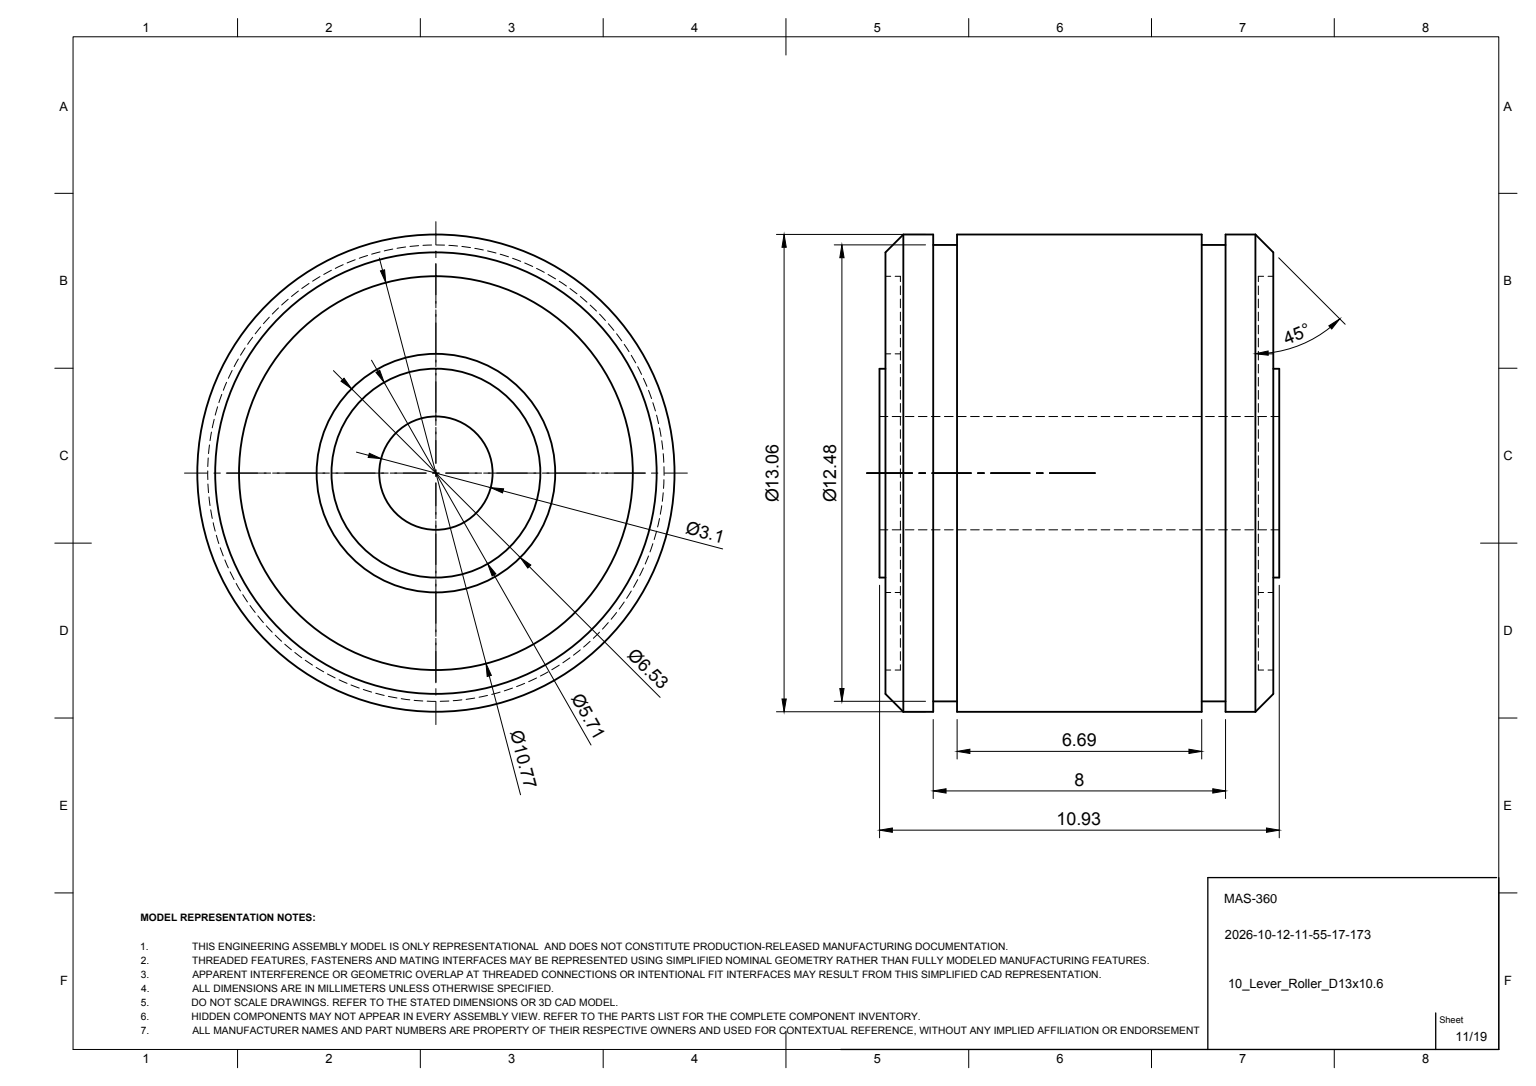
ISO-10303-21;
HEADER;
/* Generated by software containing ST-Developer
 * from STEP Tools, Inc. (www.steptools.com) 
 */

FILE_DESCRIPTION(
/* description */ (''),
/* implementation_level */ '2;1');

FILE_NAME(
/* name */ '10_Lever_Roller_D13x10.6.step',
/* time_stamp */ '2026-11-04T18:53:29-08:00',
/* author */ (''),
/* organization */ (''),
/* preprocessor_version */ 'ST-DEVELOPER v20.2',
/* originating_system */ 'Autodesk Translation Framework v15.17.0.0',
/* authorisation */ '');

FILE_SCHEMA (('AUTOMOTIVE_DESIGN { 1 0 10303 214 3 1 1 }'));
ENDSEC;

DATA;
#10=MECHANICAL_DESIGN_GEOMETRIC_PRESENTATION_REPRESENTATION('',(#1337),#100031);
#235=CONICAL_SURFACE('',#22396,6.2832,0.785398163397447);
#236=CONICAL_SURFACE('',#22400,6.2832,0.785398163397447);
#1116=CIRCLE('',#22353,2.8556);
#1117=CIRCLE('',#22354,1.55);
#1118=CIRCLE('',#22356,2.8556);
#1119=CIRCLE('',#22358,5.3856);
#1120=CIRCLE('',#22359,5.3856);
#1121=CIRCLE('',#22361,3.2636);
#1122=CIRCLE('',#22363,3.2636);
#1123=CIRCLE('',#22366,2.8556);
#1124=CIRCLE('',#22367,2.8556);
#1125=CIRCLE('',#22369,1.55);
#1126=CIRCLE('',#22371,3.2636);
#1127=CIRCLE('',#22372,3.2636);
#1128=CIRCLE('',#22374,5.3856);
#1129=CIRCLE('',#22376,5.3856);
#1130=CIRCLE('',#22378,6.0384);
#1131=CIRCLE('',#22380,6.528);
#1132=CIRCLE('',#22381,6.2424);
#1133=CIRCLE('',#22383,6.2424);
#1134=CIRCLE('',#22385,6.528);
#1135=CIRCLE('',#22387,6.528);
#1136=CIRCLE('',#22389,6.2424);
#1137=CIRCLE('',#22391,6.2424);
#1138=CIRCLE('',#22393,6.528);
#1139=CIRCLE('',#22395,6.528);
#1140=CIRCLE('',#22397,6.0384);
#1141=CIRCLE('',#22399,6.528);
#1301=SHAPE_REPRESENTATION_RELATIONSHIP('SRR','None',#100111,#1319);
#1319=ADVANCED_BREP_SHAPE_REPRESENTATION('',(#1355),#100023);
#1337=STYLED_ITEM('',(#100200),#1355);
#1355=MANIFOLD_SOLID_BREP('Body1',#20127);
#1663=PLANE('',#22352);
#1664=PLANE('',#22360);
#1665=PLANE('',#22364);
#1666=PLANE('',#22368);
#1667=PLANE('',#22373);
#1668=PLANE('',#22377);
#1669=PLANE('',#22379);
#1670=PLANE('',#22384);
#1671=PLANE('',#22388);
#1672=PLANE('',#22392);
#1673=PLANE('',#22401);
#1674=PLANE('',#22403);
#1790=FACE_BOUND('',#7364,.T.);
#1791=FACE_BOUND('',#7368,.T.);
#1792=FACE_BOUND('',#7371,.T.);
#1793=FACE_BOUND('',#7374,.T.);
#1794=FACE_BOUND('',#7377,.T.);
#1795=FACE_BOUND('',#7380,.T.);
#1796=FACE_BOUND('',#7382,.T.);
#1797=FACE_BOUND('',#7385,.T.);
#1798=FACE_BOUND('',#7388,.T.);
#1799=FACE_BOUND('',#7391,.T.);
#1800=FACE_BOUND('',#7397,.T.);
#1801=FACE_BOUND('',#7400,.T.);
#3227=LINE('',#99720,#4514);
#3228=LINE('',#99725,#4515);
#3229=LINE('',#99732,#4516);
#3230=LINE('',#99739,#4517);
#3231=LINE('',#99748,#4518);
#3232=LINE('',#99755,#4519);
#3233=LINE('',#99767,#4520);
#3234=LINE('',#99774,#4521);
#3235=LINE('',#99781,#4522);
#3236=LINE('',#99788,#4523);
#3237=LINE('',#99792,#4524);
#3238=LINE('',#99797,#4525);
#3239=LINE('',#99799,#4526);
#3240=LINE('',#99802,#4527);
#4514=VECTOR('',#27818,2.8556);
#4515=VECTOR('',#27823,5.3856);
#4516=VECTOR('',#27832,3.2636);
#4517=VECTOR('',#27841,2.8556);
#4518=VECTOR('',#27852,3.2636);
#4519=VECTOR('',#27861,5.3856);
#4520=VECTOR('',#27876,6.2424);
#4521=VECTOR('',#27885,6.528);
#4522=VECTOR('',#27894,6.2424);
#4523=VECTOR('',#27903,6.528);
#4524=VECTOR('',#27908,6.2832);
#4525=VECTOR('',#27915,6.528);
#4526=VECTOR('',#27918,6.2832);
#4527=VECTOR('',#27923,1.55);
#5001=CYLINDRICAL_SURFACE('',#22355,2.8556);
#5002=CYLINDRICAL_SURFACE('',#22357,5.3856);
#5003=CYLINDRICAL_SURFACE('',#22362,3.2636);
#5004=CYLINDRICAL_SURFACE('',#22365,2.8556);
#5005=CYLINDRICAL_SURFACE('',#22370,3.2636);
#5006=CYLINDRICAL_SURFACE('',#22375,5.3856);
#5007=CYLINDRICAL_SURFACE('',#22382,6.2424);
#5008=CYLINDRICAL_SURFACE('',#22386,6.528);
#5009=CYLINDRICAL_SURFACE('',#22390,6.2424);
#5010=CYLINDRICAL_SURFACE('',#22394,6.528);
#5011=CYLINDRICAL_SURFACE('',#22398,6.528);
#5012=CYLINDRICAL_SURFACE('',#22402,1.55);
#6110=FACE_OUTER_BOUND('',#7363,.T.);
#6111=FACE_OUTER_BOUND('',#7365,.T.);
#6112=FACE_OUTER_BOUND('',#7366,.T.);
#6113=FACE_OUTER_BOUND('',#7367,.T.);
#6114=FACE_OUTER_BOUND('',#7369,.T.);
#6115=FACE_OUTER_BOUND('',#7370,.T.);
#6116=FACE_OUTER_BOUND('',#7372,.T.);
#6117=FACE_OUTER_BOUND('',#7373,.T.);
#6118=FACE_OUTER_BOUND('',#7375,.T.);
#6119=FACE_OUTER_BOUND('',#7376,.T.);
#6120=FACE_OUTER_BOUND('',#7378,.T.);
#6121=FACE_OUTER_BOUND('',#7379,.T.);
#6122=FACE_OUTER_BOUND('',#7381,.T.);
#6123=FACE_OUTER_BOUND('',#7383,.T.);
#6124=FACE_OUTER_BOUND('',#7384,.T.);
#6125=FACE_OUTER_BOUND('',#7386,.T.);
#6126=FACE_OUTER_BOUND('',#7387,.T.);
#6127=FACE_OUTER_BOUND('',#7389,.T.);
#6128=FACE_OUTER_BOUND('',#7390,.T.);
#6129=FACE_OUTER_BOUND('',#7392,.T.);
#6130=FACE_OUTER_BOUND('',#7393,.T.);
#6131=FACE_OUTER_BOUND('',#7394,.T.);
#6132=FACE_OUTER_BOUND('',#7395,.T.);
#6133=FACE_OUTER_BOUND('',#7396,.T.);
#6134=FACE_OUTER_BOUND('',#7398,.T.);
#6135=FACE_OUTER_BOUND('',#7399,.T.);
#7363=EDGE_LOOP('',(#18635));
#7364=EDGE_LOOP('',(#18636));
#7365=EDGE_LOOP('',(#18637,#18638,#18639,#18640));
#7366=EDGE_LOOP('',(#18641,#18642,#18643,#18644));
#7367=EDGE_LOOP('',(#18645));
#7368=EDGE_LOOP('',(#18646));
#7369=EDGE_LOOP('',(#18647,#18648,#18649,#18650));
#7370=EDGE_LOOP('',(#18651));
#7371=EDGE_LOOP('',(#18652));
#7372=EDGE_LOOP('',(#18653,#18654,#18655,#18656));
#7373=EDGE_LOOP('',(#18657));
#7374=EDGE_LOOP('',(#18658));
#7375=EDGE_LOOP('',(#18659,#18660,#18661,#18662));
#7376=EDGE_LOOP('',(#18663));
#7377=EDGE_LOOP('',(#18664));
#7378=EDGE_LOOP('',(#18665,#18666,#18667,#18668));
#7379=EDGE_LOOP('',(#18669));
#7380=EDGE_LOOP('',(#18670));
#7381=EDGE_LOOP('',(#18671));
#7382=EDGE_LOOP('',(#18672));
#7383=EDGE_LOOP('',(#18673,#18674,#18675,#18676));
#7384=EDGE_LOOP('',(#18677));
#7385=EDGE_LOOP('',(#18678));
#7386=EDGE_LOOP('',(#18679,#18680,#18681,#18682));
#7387=EDGE_LOOP('',(#18683));
#7388=EDGE_LOOP('',(#18684));
#7389=EDGE_LOOP('',(#18685,#18686,#18687,#18688));
#7390=EDGE_LOOP('',(#18689));
#7391=EDGE_LOOP('',(#18690));
#7392=EDGE_LOOP('',(#18691,#18692,#18693,#18694));
#7393=EDGE_LOOP('',(#18695,#18696,#18697,#18698));
#7394=EDGE_LOOP('',(#18699,#18700,#18701,#18702));
#7395=EDGE_LOOP('',(#18703,#18704,#18705,#18706));
#7396=EDGE_LOOP('',(#18707));
#7397=EDGE_LOOP('',(#18708));
#7398=EDGE_LOOP('',(#18709,#18710,#18711,#18712));
#7399=EDGE_LOOP('',(#18713));
#7400=EDGE_LOOP('',(#18714));
#9857=VERTEX_POINT('',#99713);
#9858=VERTEX_POINT('',#99715);
#9859=VERTEX_POINT('',#99718);
#9860=VERTEX_POINT('',#99722);
#9861=VERTEX_POINT('',#99724);
#9862=VERTEX_POINT('',#99728);
#9863=VERTEX_POINT('',#99731);
#9864=VERTEX_POINT('',#99736);
#9865=VERTEX_POINT('',#99738);
#9866=VERTEX_POINT('',#99742);
#9867=VERTEX_POINT('',#99745);
#9868=VERTEX_POINT('',#99747);
#9869=VERTEX_POINT('',#99751);
#9870=VERTEX_POINT('',#99754);
#9871=VERTEX_POINT('',#99758);
#9872=VERTEX_POINT('',#99761);
#9873=VERTEX_POINT('',#99763);
#9874=VERTEX_POINT('',#99766);
#9875=VERTEX_POINT('',#99770);
#9876=VERTEX_POINT('',#99773);
#9877=VERTEX_POINT('',#99777);
#9878=VERTEX_POINT('',#99780);
#9879=VERTEX_POINT('',#99784);
#9880=VERTEX_POINT('',#99787);
#9881=VERTEX_POINT('',#99791);
#9882=VERTEX_POINT('',#99795);
#12792=EDGE_CURVE('',#9857,#9857,#1116,.T.);
#12793=EDGE_CURVE('',#9858,#9858,#1117,.T.);
#12794=EDGE_CURVE('',#9859,#9859,#1118,.T.);
#12795=EDGE_CURVE('',#9859,#9857,#3227,.T.);
#12796=EDGE_CURVE('',#9860,#9860,#1119,.T.);
#12797=EDGE_CURVE('',#9860,#9861,#3228,.T.);
#12798=EDGE_CURVE('',#9861,#9861,#1120,.T.);
#12799=EDGE_CURVE('',#9862,#9862,#1121,.T.);
#12800=EDGE_CURVE('',#9862,#9863,#3229,.T.);
#12801=EDGE_CURVE('',#9863,#9863,#1122,.T.);
#12802=EDGE_CURVE('',#9864,#9864,#1123,.T.);
#12803=EDGE_CURVE('',#9864,#9865,#3230,.T.);
#12804=EDGE_CURVE('',#9865,#9865,#1124,.T.);
#12805=EDGE_CURVE('',#9866,#9866,#1125,.T.);
#12806=EDGE_CURVE('',#9867,#9867,#1126,.T.);
#12807=EDGE_CURVE('',#9867,#9868,#3231,.T.);
#12808=EDGE_CURVE('',#9868,#9868,#1127,.T.);
#12809=EDGE_CURVE('',#9869,#9869,#1128,.T.);
#12810=EDGE_CURVE('',#9869,#9870,#3232,.T.);
#12811=EDGE_CURVE('',#9870,#9870,#1129,.T.);
#12812=EDGE_CURVE('',#9871,#9871,#1130,.T.);
#12813=EDGE_CURVE('',#9872,#9872,#1131,.T.);
#12814=EDGE_CURVE('',#9873,#9873,#1132,.T.);
#12815=EDGE_CURVE('',#9873,#9874,#3233,.T.);
#12816=EDGE_CURVE('',#9874,#9874,#1133,.T.);
#12817=EDGE_CURVE('',#9875,#9875,#1134,.T.);
#12818=EDGE_CURVE('',#9875,#9876,#3234,.T.);
#12819=EDGE_CURVE('',#9876,#9876,#1135,.T.);
#12820=EDGE_CURVE('',#9877,#9877,#1136,.T.);
#12821=EDGE_CURVE('',#9877,#9878,#3235,.T.);
#12822=EDGE_CURVE('',#9878,#9878,#1137,.T.);
#12823=EDGE_CURVE('',#9879,#9879,#1138,.T.);
#12824=EDGE_CURVE('',#9879,#9880,#3236,.T.);
#12825=EDGE_CURVE('',#9880,#9880,#1139,.T.);
#12826=EDGE_CURVE('',#9880,#9881,#3237,.T.);
#12827=EDGE_CURVE('',#9881,#9881,#1140,.T.);
#12828=EDGE_CURVE('',#9882,#9882,#1141,.T.);
#12829=EDGE_CURVE('',#9882,#9872,#3238,.T.);
#12830=EDGE_CURVE('',#9882,#9871,#3239,.T.);
#12831=EDGE_CURVE('',#9858,#9866,#3240,.T.);
#18635=ORIENTED_EDGE('',*,*,#12792,.F.);
#18636=ORIENTED_EDGE('',*,*,#12793,.T.);
#18637=ORIENTED_EDGE('',*,*,#12794,.F.);
#18638=ORIENTED_EDGE('',*,*,#12795,.T.);
#18639=ORIENTED_EDGE('',*,*,#12792,.T.);
#18640=ORIENTED_EDGE('',*,*,#12795,.F.);
#18641=ORIENTED_EDGE('',*,*,#12796,.F.);
#18642=ORIENTED_EDGE('',*,*,#12797,.T.);
#18643=ORIENTED_EDGE('',*,*,#12798,.T.);
#18644=ORIENTED_EDGE('',*,*,#12797,.F.);
#18645=ORIENTED_EDGE('',*,*,#12798,.F.);
#18646=ORIENTED_EDGE('',*,*,#12799,.T.);
#18647=ORIENTED_EDGE('',*,*,#12799,.F.);
#18648=ORIENTED_EDGE('',*,*,#12800,.T.);
#18649=ORIENTED_EDGE('',*,*,#12801,.F.);
#18650=ORIENTED_EDGE('',*,*,#12800,.F.);
#18651=ORIENTED_EDGE('',*,*,#12801,.T.);
#18652=ORIENTED_EDGE('',*,*,#12794,.T.);
#18653=ORIENTED_EDGE('',*,*,#12802,.F.);
#18654=ORIENTED_EDGE('',*,*,#12803,.T.);
#18655=ORIENTED_EDGE('',*,*,#12804,.F.);
#18656=ORIENTED_EDGE('',*,*,#12803,.F.);
#18657=ORIENTED_EDGE('',*,*,#12802,.T.);
#18658=ORIENTED_EDGE('',*,*,#12805,.F.);
#18659=ORIENTED_EDGE('',*,*,#12806,.F.);
#18660=ORIENTED_EDGE('',*,*,#12807,.T.);
#18661=ORIENTED_EDGE('',*,*,#12808,.T.);
#18662=ORIENTED_EDGE('',*,*,#12807,.F.);
#18663=ORIENTED_EDGE('',*,*,#12809,.T.);
#18664=ORIENTED_EDGE('',*,*,#12808,.F.);
#18665=ORIENTED_EDGE('',*,*,#12809,.F.);
#18666=ORIENTED_EDGE('',*,*,#12810,.T.);
#18667=ORIENTED_EDGE('',*,*,#12811,.F.);
#18668=ORIENTED_EDGE('',*,*,#12810,.F.);
#18669=ORIENTED_EDGE('',*,*,#12812,.T.);
#18670=ORIENTED_EDGE('',*,*,#12811,.T.);
#18671=ORIENTED_EDGE('',*,*,#12813,.F.);
#18672=ORIENTED_EDGE('',*,*,#12814,.T.);
#18673=ORIENTED_EDGE('',*,*,#12814,.F.);
#18674=ORIENTED_EDGE('',*,*,#12815,.T.);
#18675=ORIENTED_EDGE('',*,*,#12816,.T.);
#18676=ORIENTED_EDGE('',*,*,#12815,.F.);
#18677=ORIENTED_EDGE('',*,*,#12817,.F.);
#18678=ORIENTED_EDGE('',*,*,#12816,.F.);
#18679=ORIENTED_EDGE('',*,*,#12817,.T.);
#18680=ORIENTED_EDGE('',*,*,#12818,.T.);
#18681=ORIENTED_EDGE('',*,*,#12819,.T.);
#18682=ORIENTED_EDGE('',*,*,#12818,.F.);
#18683=ORIENTED_EDGE('',*,*,#12819,.F.);
#18684=ORIENTED_EDGE('',*,*,#12820,.T.);
#18685=ORIENTED_EDGE('',*,*,#12820,.F.);
#18686=ORIENTED_EDGE('',*,*,#12821,.T.);
#18687=ORIENTED_EDGE('',*,*,#12822,.T.);
#18688=ORIENTED_EDGE('',*,*,#12821,.F.);
#18689=ORIENTED_EDGE('',*,*,#12823,.F.);
#18690=ORIENTED_EDGE('',*,*,#12822,.F.);
#18691=ORIENTED_EDGE('',*,*,#12823,.T.);
#18692=ORIENTED_EDGE('',*,*,#12824,.T.);
#18693=ORIENTED_EDGE('',*,*,#12825,.T.);
#18694=ORIENTED_EDGE('',*,*,#12824,.F.);
#18695=ORIENTED_EDGE('',*,*,#12825,.F.);
#18696=ORIENTED_EDGE('',*,*,#12826,.T.);
#18697=ORIENTED_EDGE('',*,*,#12827,.T.);
#18698=ORIENTED_EDGE('',*,*,#12826,.F.);
#18699=ORIENTED_EDGE('',*,*,#12828,.F.);
#18700=ORIENTED_EDGE('',*,*,#12829,.T.);
#18701=ORIENTED_EDGE('',*,*,#12813,.T.);
#18702=ORIENTED_EDGE('',*,*,#12829,.F.);
#18703=ORIENTED_EDGE('',*,*,#12828,.T.);
#18704=ORIENTED_EDGE('',*,*,#12830,.T.);
#18705=ORIENTED_EDGE('',*,*,#12812,.F.);
#18706=ORIENTED_EDGE('',*,*,#12830,.F.);
#18707=ORIENTED_EDGE('',*,*,#12806,.T.);
#18708=ORIENTED_EDGE('',*,*,#12804,.T.);
#18709=ORIENTED_EDGE('',*,*,#12793,.F.);
#18710=ORIENTED_EDGE('',*,*,#12831,.T.);
#18711=ORIENTED_EDGE('',*,*,#12805,.T.);
#18712=ORIENTED_EDGE('',*,*,#12831,.F.);
#18713=ORIENTED_EDGE('',*,*,#12827,.F.);
#18714=ORIENTED_EDGE('',*,*,#12796,.T.);
#20044=ADVANCED_FACE('',(#6110,#1790),#1663,.T.);
#20045=ADVANCED_FACE('',(#6111),#5001,.T.);
#20046=ADVANCED_FACE('',(#6112),#5002,.F.);
#20047=ADVANCED_FACE('',(#6113,#1791),#1664,.F.);
#20048=ADVANCED_FACE('',(#6114),#5003,.T.);
#20049=ADVANCED_FACE('',(#6115,#1792),#1665,.T.);
#20050=ADVANCED_FACE('',(#6116),#5004,.T.);
#20051=ADVANCED_FACE('',(#6117,#1793),#1666,.T.);
#20052=ADVANCED_FACE('',(#6118),#5005,.T.);
#20053=ADVANCED_FACE('',(#6119,#1794),#1667,.F.);
#20054=ADVANCED_FACE('',(#6120),#5006,.F.);
#20055=ADVANCED_FACE('',(#6121,#1795),#1668,.T.);
#20056=ADVANCED_FACE('',(#6122,#1796),#1669,.F.);
#20057=ADVANCED_FACE('',(#6123),#5007,.T.);
#20058=ADVANCED_FACE('',(#6124,#1797),#1670,.F.);
#20059=ADVANCED_FACE('',(#6125),#5008,.T.);
#20060=ADVANCED_FACE('',(#6126,#1798),#1671,.F.);
#20061=ADVANCED_FACE('',(#6127),#5009,.T.);
#20062=ADVANCED_FACE('',(#6128,#1799),#1672,.F.);
#20063=ADVANCED_FACE('',(#6129),#5010,.T.);
#20064=ADVANCED_FACE('',(#6130),#235,.T.);
#20065=ADVANCED_FACE('',(#6131),#5011,.T.);
#20066=ADVANCED_FACE('',(#6132),#236,.T.);
#20067=ADVANCED_FACE('',(#6133,#1800),#1673,.T.);
#20068=ADVANCED_FACE('',(#6134),#5012,.F.);
#20069=ADVANCED_FACE('',(#6135,#1801),#1674,.T.);
#20127=CLOSED_SHELL('',(#20044,#20045,#20046,#20047,#20048,#20049,#20050,
#20051,#20052,#20053,#20054,#20055,#20056,#20057,#20058,#20059,#20060,#20061,
#20062,#20063,#20064,#20065,#20066,#20067,#20068,#20069));
#22351=AXIS2_PLACEMENT_3D('',#99711,#27806,#27807);
#22352=AXIS2_PLACEMENT_3D('',#99712,#27808,#27809);
#22353=AXIS2_PLACEMENT_3D('',#99714,#27810,#27811);
#22354=AXIS2_PLACEMENT_3D('',#99716,#27812,#27813);
#22355=AXIS2_PLACEMENT_3D('',#99717,#27814,#27815);
#22356=AXIS2_PLACEMENT_3D('',#99719,#27816,#27817);
#22357=AXIS2_PLACEMENT_3D('',#99721,#27819,#27820);
#22358=AXIS2_PLACEMENT_3D('',#99723,#27821,#27822);
#22359=AXIS2_PLACEMENT_3D('',#99726,#27824,#27825);
#22360=AXIS2_PLACEMENT_3D('',#99727,#27826,#27827);
#22361=AXIS2_PLACEMENT_3D('',#99729,#27828,#27829);
#22362=AXIS2_PLACEMENT_3D('',#99730,#27830,#27831);
#22363=AXIS2_PLACEMENT_3D('',#99733,#27833,#27834);
#22364=AXIS2_PLACEMENT_3D('',#99734,#27835,#27836);
#22365=AXIS2_PLACEMENT_3D('',#99735,#27837,#27838);
#22366=AXIS2_PLACEMENT_3D('',#99737,#27839,#27840);
#22367=AXIS2_PLACEMENT_3D('',#99740,#27842,#27843);
#22368=AXIS2_PLACEMENT_3D('',#99741,#27844,#27845);
#22369=AXIS2_PLACEMENT_3D('',#99743,#27846,#27847);
#22370=AXIS2_PLACEMENT_3D('',#99744,#27848,#27849);
#22371=AXIS2_PLACEMENT_3D('',#99746,#27850,#27851);
#22372=AXIS2_PLACEMENT_3D('',#99749,#27853,#27854);
#22373=AXIS2_PLACEMENT_3D('',#99750,#27855,#27856);
#22374=AXIS2_PLACEMENT_3D('',#99752,#27857,#27858);
#22375=AXIS2_PLACEMENT_3D('',#99753,#27859,#27860);
#22376=AXIS2_PLACEMENT_3D('',#99756,#27862,#27863);
#22377=AXIS2_PLACEMENT_3D('',#99757,#27864,#27865);
#22378=AXIS2_PLACEMENT_3D('',#99759,#27866,#27867);
#22379=AXIS2_PLACEMENT_3D('',#99760,#27868,#27869);
#22380=AXIS2_PLACEMENT_3D('',#99762,#27870,#27871);
#22381=AXIS2_PLACEMENT_3D('',#99764,#27872,#27873);
#22382=AXIS2_PLACEMENT_3D('',#99765,#27874,#27875);
#22383=AXIS2_PLACEMENT_3D('',#99768,#27877,#27878);
#22384=AXIS2_PLACEMENT_3D('',#99769,#27879,#27880);
#22385=AXIS2_PLACEMENT_3D('',#99771,#27881,#27882);
#22386=AXIS2_PLACEMENT_3D('',#99772,#27883,#27884);
#22387=AXIS2_PLACEMENT_3D('',#99775,#27886,#27887);
#22388=AXIS2_PLACEMENT_3D('',#99776,#27888,#27889);
#22389=AXIS2_PLACEMENT_3D('',#99778,#27890,#27891);
#22390=AXIS2_PLACEMENT_3D('',#99779,#27892,#27893);
#22391=AXIS2_PLACEMENT_3D('',#99782,#27895,#27896);
#22392=AXIS2_PLACEMENT_3D('',#99783,#27897,#27898);
#22393=AXIS2_PLACEMENT_3D('',#99785,#27899,#27900);
#22394=AXIS2_PLACEMENT_3D('',#99786,#27901,#27902);
#22395=AXIS2_PLACEMENT_3D('',#99789,#27904,#27905);
#22396=AXIS2_PLACEMENT_3D('',#99790,#27906,#27907);
#22397=AXIS2_PLACEMENT_3D('',#99793,#27909,#27910);
#22398=AXIS2_PLACEMENT_3D('',#99794,#27911,#27912);
#22399=AXIS2_PLACEMENT_3D('',#99796,#27913,#27914);
#22400=AXIS2_PLACEMENT_3D('',#99798,#27916,#27917);
#22401=AXIS2_PLACEMENT_3D('',#99800,#27919,#27920);
#22402=AXIS2_PLACEMENT_3D('',#99801,#27921,#27922);
#22403=AXIS2_PLACEMENT_3D('',#99803,#27924,#27925);
#27806=DIRECTION('axis',(0.,0.,1.));
#27807=DIRECTION('refdir',(1.,0.,0.));
#27808=DIRECTION('center_axis',(-1.,0.,0.));
#27809=DIRECTION('ref_axis',(0.,0.,1.));
#27810=DIRECTION('center_axis',(1.,0.,0.));
#27811=DIRECTION('ref_axis',(0.,0.,-1.));
#27812=DIRECTION('center_axis',(1.,0.,0.));
#27813=DIRECTION('ref_axis',(0.,0.,-1.));
#27814=DIRECTION('center_axis',(1.,0.,0.));
#27815=DIRECTION('ref_axis',(0.,1.,0.));
#27816=DIRECTION('center_axis',(1.,0.,0.));
#27817=DIRECTION('ref_axis',(0.,1.,0.));
#27818=DIRECTION('',(-1.,0.,0.));
#27819=DIRECTION('center_axis',(1.,0.,0.));
#27820=DIRECTION('ref_axis',(0.,1.,0.));
#27821=DIRECTION('center_axis',(1.,0.,0.));
#27822=DIRECTION('ref_axis',(0.,1.,0.));
#27823=DIRECTION('',(1.,0.,0.));
#27824=DIRECTION('center_axis',(1.,0.,0.));
#27825=DIRECTION('ref_axis',(0.,0.,-1.));
#27826=DIRECTION('center_axis',(1.,0.,0.));
#27827=DIRECTION('ref_axis',(0.,0.,-1.));
#27828=DIRECTION('center_axis',(1.,0.,0.));
#27829=DIRECTION('ref_axis',(0.,0.,-1.));
#27830=DIRECTION('center_axis',(1.,0.,0.));
#27831=DIRECTION('ref_axis',(0.,1.,0.));
#27832=DIRECTION('',(-1.,0.,0.));
#27833=DIRECTION('center_axis',(-1.,0.,0.));
#27834=DIRECTION('ref_axis',(0.,1.,0.));
#27835=DIRECTION('center_axis',(-1.,0.,0.));
#27836=DIRECTION('ref_axis',(0.,0.,1.));
#27837=DIRECTION('center_axis',(1.,0.,0.));
#27838=DIRECTION('ref_axis',(0.,1.,0.));
#27839=DIRECTION('center_axis',(1.,0.,0.));
#27840=DIRECTION('ref_axis',(0.,0.,-1.));
#27841=DIRECTION('',(-1.,0.,0.));
#27842=DIRECTION('center_axis',(-1.,0.,0.));
#27843=DIRECTION('ref_axis',(0.,1.,0.));
#27844=DIRECTION('center_axis',(1.,0.,0.));
#27845=DIRECTION('ref_axis',(0.,0.,-1.));
#27846=DIRECTION('center_axis',(1.,0.,0.));
#27847=DIRECTION('ref_axis',(0.,0.,-1.));
#27848=DIRECTION('center_axis',(1.,0.,0.));
#27849=DIRECTION('ref_axis',(0.,1.,0.));
#27850=DIRECTION('center_axis',(1.,0.,0.));
#27851=DIRECTION('ref_axis',(0.,1.,0.));
#27852=DIRECTION('',(-1.,0.,0.));
#27853=DIRECTION('center_axis',(1.,0.,0.));
#27854=DIRECTION('ref_axis',(0.,0.,-1.));
#27855=DIRECTION('center_axis',(-1.,0.,0.));
#27856=DIRECTION('ref_axis',(0.,0.,1.));
#27857=DIRECTION('center_axis',(1.,0.,0.));
#27858=DIRECTION('ref_axis',(0.,0.,-1.));
#27859=DIRECTION('center_axis',(1.,0.,0.));
#27860=DIRECTION('ref_axis',(0.,1.,0.));
#27861=DIRECTION('',(1.,0.,0.));
#27862=DIRECTION('center_axis',(-1.,0.,0.));
#27863=DIRECTION('ref_axis',(0.,1.,0.));
#27864=DIRECTION('center_axis',(1.,0.,0.));
#27865=DIRECTION('ref_axis',(0.,0.,-1.));
#27866=DIRECTION('center_axis',(1.,0.,0.));
#27867=DIRECTION('ref_axis',(0.,0.,-1.));
#27868=DIRECTION('center_axis',(1.,0.,0.));
#27869=DIRECTION('ref_axis',(0.,0.,-1.));
#27870=DIRECTION('center_axis',(1.,0.,0.));
#27871=DIRECTION('ref_axis',(0.,1.,0.));
#27872=DIRECTION('center_axis',(1.,0.,0.));
#27873=DIRECTION('ref_axis',(0.,0.,-1.));
#27874=DIRECTION('center_axis',(1.,0.,0.));
#27875=DIRECTION('ref_axis',(0.,1.,0.));
#27876=DIRECTION('',(-1.,0.,0.));
#27877=DIRECTION('center_axis',(1.,0.,0.));
#27878=DIRECTION('ref_axis',(0.,0.,-1.));
#27879=DIRECTION('center_axis',(-1.,0.,0.));
#27880=DIRECTION('ref_axis',(0.,0.,1.));
#27881=DIRECTION('center_axis',(-1.,0.,0.));
#27882=DIRECTION('ref_axis',(0.,1.,0.));
#27883=DIRECTION('center_axis',(1.,0.,0.));
#27884=DIRECTION('ref_axis',(0.,1.,0.));
#27885=DIRECTION('',(-1.,0.,0.));
#27886=DIRECTION('center_axis',(1.,0.,0.));
#27887=DIRECTION('ref_axis',(0.,1.,0.));
#27888=DIRECTION('center_axis',(1.,0.,0.));
#27889=DIRECTION('ref_axis',(0.,0.,-1.));
#27890=DIRECTION('center_axis',(1.,0.,0.));
#27891=DIRECTION('ref_axis',(0.,0.,-1.));
#27892=DIRECTION('center_axis',(1.,0.,0.));
#27893=DIRECTION('ref_axis',(0.,1.,0.));
#27894=DIRECTION('',(-1.,0.,0.));
#27895=DIRECTION('center_axis',(1.,0.,0.));
#27896=DIRECTION('ref_axis',(0.,0.,-1.));
#27897=DIRECTION('center_axis',(-1.,0.,0.));
#27898=DIRECTION('ref_axis',(0.,0.,1.));
#27899=DIRECTION('center_axis',(-1.,0.,0.));
#27900=DIRECTION('ref_axis',(0.,1.,0.));
#27901=DIRECTION('center_axis',(1.,0.,0.));
#27902=DIRECTION('ref_axis',(0.,1.,0.));
#27903=DIRECTION('',(-1.,0.,0.));
#27904=DIRECTION('center_axis',(1.,0.,0.));
#27905=DIRECTION('ref_axis',(0.,0.,-1.));
#27906=DIRECTION('center_axis',(1.,0.,0.));
#27907=DIRECTION('ref_axis',(0.,1.,0.));
#27908=DIRECTION('',(-0.707106781186548,0.707106781186547,8.65956056235492E-17));
#27909=DIRECTION('center_axis',(1.,0.,0.));
#27910=DIRECTION('ref_axis',(0.,0.,-1.));
#27911=DIRECTION('center_axis',(1.,0.,0.));
#27912=DIRECTION('ref_axis',(0.,1.,0.));
#27913=DIRECTION('center_axis',(1.,0.,0.));
#27914=DIRECTION('ref_axis',(0.,0.,-1.));
#27915=DIRECTION('',(-1.,0.,0.));
#27916=DIRECTION('center_axis',(-1.,0.,0.));
#27917=DIRECTION('ref_axis',(0.,1.,0.));
#27918=DIRECTION('',(0.707106781186548,0.707106781186547,-8.65956056235492E-17));
#27919=DIRECTION('center_axis',(1.,0.,0.));
#27920=DIRECTION('ref_axis',(0.,0.,-1.));
#27921=DIRECTION('center_axis',(1.,0.,0.));
#27922=DIRECTION('ref_axis',(0.,1.,0.));
#27923=DIRECTION('',(1.,0.,0.));
#27924=DIRECTION('center_axis',(-1.,0.,0.));
#27925=DIRECTION('ref_axis',(0.,0.,1.));
#99711=CARTESIAN_POINT('',(0.,0.,0.));
#99712=CARTESIAN_POINT('Origin',(-5.4672,2.8556,0.));
#99713=CARTESIAN_POINT('',(-5.4672,-2.8556,-3.49710139964518E-16));
#99714=CARTESIAN_POINT('Origin',(-5.4672,0.,0.));
#99715=CARTESIAN_POINT('',(-5.4672,-1.55,-1.8982025386784E-16));
#99716=CARTESIAN_POINT('Origin',(-5.4672,0.,0.));
#99717=CARTESIAN_POINT('Origin',(-5.3856,0.,0.));
#99718=CARTESIAN_POINT('',(-5.304,-2.8556,-3.49710139964518E-16));
#99719=CARTESIAN_POINT('Origin',(-5.304,0.,0.));
#99720=CARTESIAN_POINT('',(-5.3856,-2.8556,-3.49710139964518E-16));
#99721=CARTESIAN_POINT('Origin',(-5.1,0.,0.));
#99722=CARTESIAN_POINT('',(-5.304,-5.3856,-6.59545780148798E-16));
#99723=CARTESIAN_POINT('Origin',(-5.304,0.,0.));
#99724=CARTESIAN_POINT('',(-4.896,-5.3856,-6.59545780148798E-16));
#99725=CARTESIAN_POINT('',(-5.1,-5.3856,-6.59545780148799E-16));
#99726=CARTESIAN_POINT('Origin',(-4.896,0.,0.));
#99727=CARTESIAN_POINT('Origin',(-4.896,3.2636,0.));
#99728=CARTESIAN_POINT('',(-4.896,-3.2636,-3.9967572936973E-16));
#99729=CARTESIAN_POINT('Origin',(-4.896,0.,0.));
#99730=CARTESIAN_POINT('Origin',(-5.1,0.,0.));
#99731=CARTESIAN_POINT('',(-5.304,-3.2636,-3.9967572936973E-16));
#99732=CARTESIAN_POINT('',(-5.1,-3.2636,-3.9967572936973E-16));
#99733=CARTESIAN_POINT('Origin',(-5.304,0.,0.));
#99734=CARTESIAN_POINT('Origin',(-5.304,6.0384,0.));
#99735=CARTESIAN_POINT('Origin',(5.3856,0.,0.));
#99736=CARTESIAN_POINT('',(5.4672,-2.8556,-3.49710139964518E-16));
#99737=CARTESIAN_POINT('Origin',(5.4672,0.,0.));
#99738=CARTESIAN_POINT('',(5.304,-2.8556,-3.49710139964518E-16));
#99739=CARTESIAN_POINT('',(5.3856,-2.8556,-3.49710139964518E-16));
#99740=CARTESIAN_POINT('Origin',(5.304,0.,0.));
#99741=CARTESIAN_POINT('Origin',(5.4672,1.55,0.));
#99742=CARTESIAN_POINT('',(5.4672,-1.55,-1.8982025386784E-16));
#99743=CARTESIAN_POINT('Origin',(5.4672,0.,0.));
#99744=CARTESIAN_POINT('Origin',(5.1,0.,0.));
#99745=CARTESIAN_POINT('',(5.304,-3.2636,-3.9967572936973E-16));
#99746=CARTESIAN_POINT('Origin',(5.304,0.,0.));
#99747=CARTESIAN_POINT('',(4.896,-3.2636,-3.9967572936973E-16));
#99748=CARTESIAN_POINT('',(5.1,-3.2636,-3.9967572936973E-16));
#99749=CARTESIAN_POINT('Origin',(4.896,0.,0.));
#99750=CARTESIAN_POINT('Origin',(4.896,5.3856,0.));
#99751=CARTESIAN_POINT('',(4.896,-5.3856,-6.59545780148798E-16));
#99752=CARTESIAN_POINT('Origin',(4.896,0.,0.));
#99753=CARTESIAN_POINT('Origin',(5.1,0.,0.));
#99754=CARTESIAN_POINT('',(5.304,-5.3856,-6.59545780148798E-16));
#99755=CARTESIAN_POINT('',(5.1,-5.3856,-6.59545780148799E-16));
#99756=CARTESIAN_POINT('Origin',(5.304,0.,0.));
#99757=CARTESIAN_POINT('Origin',(5.304,1.55,0.));
#99758=CARTESIAN_POINT('',(5.304,-6.0384,-7.39490723197138E-16));
#99759=CARTESIAN_POINT('Origin',(5.304,0.,0.));
#99760=CARTESIAN_POINT('Origin',(3.9984,6.2424,0.));
#99761=CARTESIAN_POINT('',(3.9984,-6.528,-7.99449430483392E-16));
#99762=CARTESIAN_POINT('Origin',(3.9984,0.,0.));
#99763=CARTESIAN_POINT('',(3.9984,-6.2424,-7.64473517899744E-16));
#99764=CARTESIAN_POINT('Origin',(3.9984,0.,0.));
#99765=CARTESIAN_POINT('Origin',(3.672,0.,0.));
#99766=CARTESIAN_POINT('',(3.3456,-6.2424,-7.64473517899744E-16));
#99767=CARTESIAN_POINT('',(3.672,-6.2424,-7.64473517899744E-16));
#99768=CARTESIAN_POINT('Origin',(3.3456,0.,0.));
#99769=CARTESIAN_POINT('Origin',(3.3456,6.936,0.));
#99770=CARTESIAN_POINT('',(3.3456,-6.528,7.99449430483392E-16));
#99771=CARTESIAN_POINT('Origin',(3.3456,0.,0.));
#99772=CARTESIAN_POINT('Origin',(0.,0.,0.));
#99773=CARTESIAN_POINT('',(-3.3456,-6.528,-7.99449430483392E-16));
#99774=CARTESIAN_POINT('',(0.,-6.528,-7.99449430483392E-16));
#99775=CARTESIAN_POINT('Origin',(-3.3456,0.,0.));
#99776=CARTESIAN_POINT('Origin',(-3.3456,6.2424,0.));
#99777=CARTESIAN_POINT('',(-3.3456,-6.2424,-7.64473517899744E-16));
#99778=CARTESIAN_POINT('Origin',(-3.3456,0.,0.));
#99779=CARTESIAN_POINT('Origin',(-3.672,0.,0.));
#99780=CARTESIAN_POINT('',(-3.9984,-6.2424,-7.64473517899744E-16));
#99781=CARTESIAN_POINT('',(-3.672,-6.2424,-7.64473517899744E-16));
#99782=CARTESIAN_POINT('Origin',(-3.9984,0.,0.));
#99783=CARTESIAN_POINT('Origin',(-3.9984,6.936,0.));
#99784=CARTESIAN_POINT('',(-3.9984,-6.528,7.99449430483392E-16));
#99785=CARTESIAN_POINT('Origin',(-3.9984,0.,0.));
#99786=CARTESIAN_POINT('Origin',(0.,0.,0.));
#99787=CARTESIAN_POINT('',(-4.8144,-6.528,-7.99449430483392E-16));
#99788=CARTESIAN_POINT('',(0.,-6.528,-7.99449430483392E-16));
#99789=CARTESIAN_POINT('Origin',(-4.8144,0.,0.));
#99790=CARTESIAN_POINT('Origin',(-5.0592,0.,0.));
#99791=CARTESIAN_POINT('',(-5.304,-6.0384,-7.39490723197138E-16));
#99792=CARTESIAN_POINT('',(-5.0592,-6.2832,-7.69470076840265E-16));
#99793=CARTESIAN_POINT('Origin',(-5.304,0.,0.));
#99794=CARTESIAN_POINT('Origin',(0.,0.,0.));
#99795=CARTESIAN_POINT('',(4.8144,-6.528,-7.99449430483392E-16));
#99796=CARTESIAN_POINT('Origin',(4.8144,0.,0.));
#99797=CARTESIAN_POINT('',(0.,-6.528,-7.99449430483392E-16));
#99798=CARTESIAN_POINT('Origin',(5.0592,0.,0.));
#99799=CARTESIAN_POINT('',(5.0592,-6.2832,7.69470076840265E-16));
#99800=CARTESIAN_POINT('Origin',(5.304,1.55,0.));
#99801=CARTESIAN_POINT('Origin',(0.,0.,0.));
#99802=CARTESIAN_POINT('',(0.,-1.55,-1.8982025386784E-16));
#99803=CARTESIAN_POINT('Origin',(-5.304,6.0384,0.));
#100003=UNCERTAINTY_MEASURE_WITH_UNIT(LENGTH_MEASURE(0.01),#100032,
'DISTANCE_ACCURACY_VALUE',
'Maximum model space distance between geometric entities at asserted c
onnectivities');
#100011=UNCERTAINTY_MEASURE_WITH_UNIT(LENGTH_MEASURE(0.01),#100032,
'DISTANCE_ACCURACY_VALUE',
'Maximum model space distance between geometric entities at asserted c
onnectivities');
#100023=(
GEOMETRIC_REPRESENTATION_CONTEXT(3)
GLOBAL_UNCERTAINTY_ASSIGNED_CONTEXT((#100003))
GLOBAL_UNIT_ASSIGNED_CONTEXT((#100032,#100034,#100035))
REPRESENTATION_CONTEXT('','3D')
);
#100031=(
GEOMETRIC_REPRESENTATION_CONTEXT(3)
GLOBAL_UNCERTAINTY_ASSIGNED_CONTEXT((#100011))
GLOBAL_UNIT_ASSIGNED_CONTEXT((#100032,#100034,#100035))
REPRESENTATION_CONTEXT('','3D')
);
#100032=(
LENGTH_UNIT()
NAMED_UNIT(*)
SI_UNIT(.MILLI.,.METRE.)
);
#100034=(
NAMED_UNIT(*)
PLANE_ANGLE_UNIT()
SI_UNIT($,.RADIAN.)
);
#100035=(
NAMED_UNIT(*)
SI_UNIT($,.STERADIAN.)
SOLID_ANGLE_UNIT()
);
#100047=SHAPE_DEFINITION_REPRESENTATION(#100066,#100111);
#100066=PRODUCT_DEFINITION_SHAPE('',$,#100131);
#100111=SHAPE_REPRESENTATION('',(#22351),#100023);
#100119=PRODUCT_DEFINITION_CONTEXT('part definition',#100178,'design');
#100131=PRODUCT_DEFINITION('2026-10-12-11-55-17-173',
'10_Lever_Roller_D13x10.6',#100150,#100119);
#100150=PRODUCT_DEFINITION_FORMATION('',$,#100191);
#100178=APPLICATION_CONTEXT(
'Core Data for Automotive Mechanical Design Process');
#100179=PRODUCT_CONTEXT('part definition',#100178,'mechanical');
#100191=PRODUCT('2026-10-12-11-55-17-173','10_Lever_Roller_D13x10.6',$,
(#100179));
#100200=PRESENTATION_STYLE_ASSIGNMENT((#100206));
#100206=SURFACE_STYLE_USAGE(.BOTH.,#100212);
#100212=SURFACE_SIDE_STYLE('',(#100218));
#100218=SURFACE_STYLE_FILL_AREA(#100224);
#100224=FILL_AREA_STYLE('Opaque(227,224,212)',(#100230));
#100230=FILL_AREA_STYLE_COLOUR('Opaque(227,224,212)',#100236);
#100236=COLOUR_RGB('Opaque(227,224,212)',0.890196078431372,0.87843137254902,
0.831372549019608);
ENDSEC;
END-ISO-10303-21;
